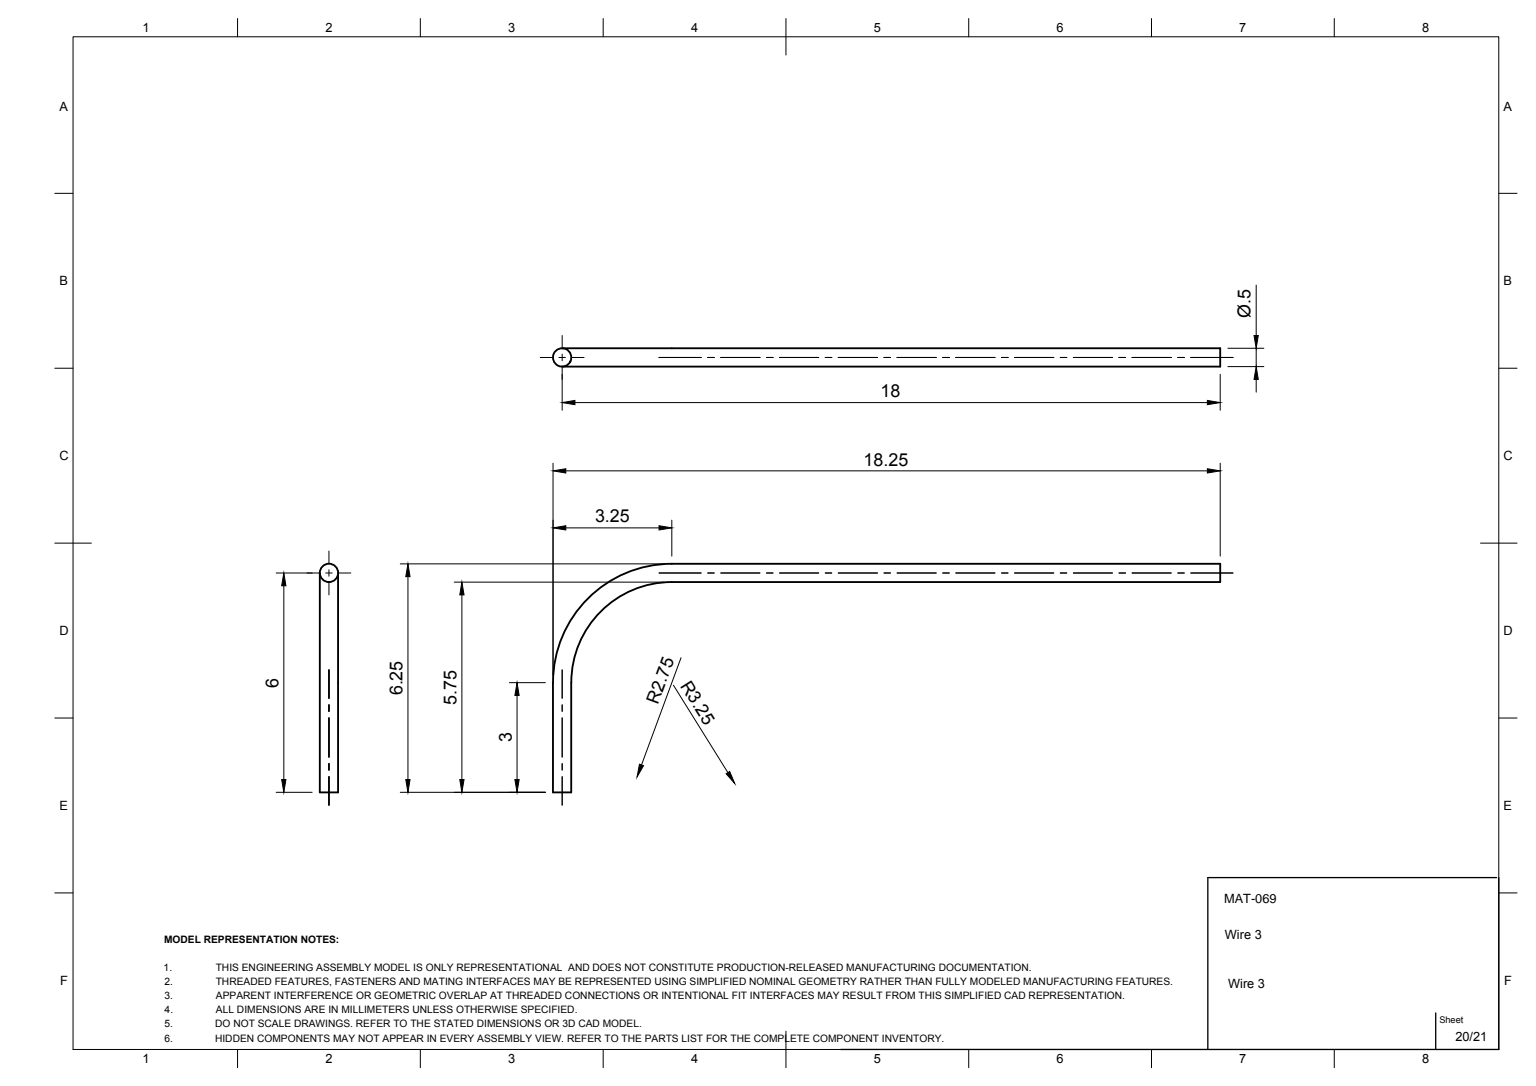
ISO-10303-21;
HEADER;
/* Generated by software containing ST-Developer
 * from STEP Tools, Inc. (www.steptools.com) 
 */

FILE_DESCRIPTION(
/* description */ ('CAx-IF Rec.Pracs.---Representation and Presentation of Product Manufa
cturing Information (PMI)---4.0---2014-10-13'),
/* implementation_level */ '2;1');

FILE_NAME(
/* name */ 'Wire 3.step',
/* time_stamp */ '2026-10-24T15:08:39-07:00',
/* author */ (''),
/* organization */ (''),
/* preprocessor_version */ 'ST-DEVELOPER v20.2',
/* originating_system */ 'Autodesk Translation Framework v15.17.0.0',
/* authorisation */ '');

FILE_SCHEMA (('AP242_MANAGED_MODEL_BASED_3D_ENGINEERING_MIM_LF { 1 0 10303 442 2 1 4 }'));
ENDSEC;

DATA;
#10=MECHANICAL_DESIGN_GEOMETRIC_PRESENTATION_REPRESENTATION('',(#838),#50081);
#779=TOROIDAL_SURFACE('',#10984,0.003,0.00025);
#798=SHAPE_REPRESENTATION_RELATIONSHIP('SRR','None',#50166,#818);
#818=ADVANCED_BREP_SHAPE_REPRESENTATION('',(#858),#50079);
#838=STYLED_ITEM('',(#50260),#858);
#858=MANIFOLD_SOLID_BREP('Body1',#9883);
#1097=PLANE('',#10990);
#1098=PLANE('',#10991);
#1625=FACE_OUTER_BOUND('',#2223,.T.);
#1626=FACE_OUTER_BOUND('',#2224,.T.);
#1627=FACE_OUTER_BOUND('',#2225,.T.);
#1628=FACE_OUTER_BOUND('',#2226,.T.);
#1629=FACE_OUTER_BOUND('',#2227,.T.);
#2223=EDGE_LOOP('',(#9060,#9061,#9062,#9063,#9064));
#2224=EDGE_LOOP('',(#9065,#9066,#9067,#9068,#9069,#9070));
#2225=EDGE_LOOP('',(#9071,#9072,#9073,#9074,#9075));
#2226=EDGE_LOOP('',(#9076));
#2227=EDGE_LOOP('',(#9077));
#2813=LINE('',#49284,#3391);
#2814=LINE('',#49296,#3392);
#3391=VECTOR('',#13357,0.00025);
#3392=VECTOR('',#13372,0.00025);
#3754=CIRCLE('',#10981,0.00025000000001);
#3755=CIRCLE('',#10982,0.00025000000001);
#3756=CIRCLE('',#10983,0.00025000000001);
#3757=CIRCLE('',#10985,0.00275);
#3758=CIRCLE('',#10986,0.00025000000001);
#3759=CIRCLE('',#10987,0.00025000000001);
#3760=CIRCLE('',#10989,0.00025000000001);
#4737=VERTEX_POINT('',#49281);
#4738=VERTEX_POINT('',#49283);
#4739=VERTEX_POINT('',#49285);
#4740=VERTEX_POINT('',#49289);
#4741=VERTEX_POINT('',#49291);
#4742=VERTEX_POINT('',#49295);
#6183=EDGE_CURVE('',#4737,#4737,#3754,.T.);
#6184=EDGE_CURVE('',#4737,#4738,#2813,.T.);
#6185=EDGE_CURVE('',#4738,#4739,#3755,.T.);
#6186=EDGE_CURVE('',#4739,#4738,#3756,.T.);
#6187=EDGE_CURVE('',#4739,#4740,#3757,.T.);
#6188=EDGE_CURVE('',#4740,#4741,#3758,.T.);
#6189=EDGE_CURVE('',#4741,#4740,#3759,.T.);
#6190=EDGE_CURVE('',#4741,#4742,#2814,.T.);
#6191=EDGE_CURVE('',#4742,#4742,#3760,.T.);
#9060=ORIENTED_EDGE('',*,*,#6183,.F.);
#9061=ORIENTED_EDGE('',*,*,#6184,.T.);
#9062=ORIENTED_EDGE('',*,*,#6185,.T.);
#9063=ORIENTED_EDGE('',*,*,#6186,.T.);
#9064=ORIENTED_EDGE('',*,*,#6184,.F.);
#9065=ORIENTED_EDGE('',*,*,#6186,.F.);
#9066=ORIENTED_EDGE('',*,*,#6187,.T.);
#9067=ORIENTED_EDGE('',*,*,#6188,.T.);
#9068=ORIENTED_EDGE('',*,*,#6189,.T.);
#9069=ORIENTED_EDGE('',*,*,#6187,.F.);
#9070=ORIENTED_EDGE('',*,*,#6185,.F.);
#9071=ORIENTED_EDGE('',*,*,#6189,.F.);
#9072=ORIENTED_EDGE('',*,*,#6190,.T.);
#9073=ORIENTED_EDGE('',*,*,#6191,.T.);
#9074=ORIENTED_EDGE('',*,*,#6190,.F.);
#9075=ORIENTED_EDGE('',*,*,#6188,.F.);
#9076=ORIENTED_EDGE('',*,*,#6183,.T.);
#9077=ORIENTED_EDGE('',*,*,#6191,.F.);
#9317=CYLINDRICAL_SURFACE('',#10980,0.00025);
#9318=CYLINDRICAL_SURFACE('',#10988,0.00025);
#9847=ADVANCED_FACE('',(#1625),#9317,.T.);
#9848=ADVANCED_FACE('',(#1626),#779,.T.);
#9849=ADVANCED_FACE('',(#1627),#9318,.T.);
#9850=ADVANCED_FACE('',(#1628),#1097,.T.);
#9851=ADVANCED_FACE('',(#1629),#1098,.F.);
#9883=CLOSED_SHELL('',(#9847,#9848,#9849,#9850,#9851));
#10979=AXIS2_PLACEMENT_3D('',#49279,#13351,#13352);
#10980=AXIS2_PLACEMENT_3D('',#49280,#13353,#13354);
#10981=AXIS2_PLACEMENT_3D('',#49282,#13355,#13356);
#10982=AXIS2_PLACEMENT_3D('',#49286,#13358,#13359);
#10983=AXIS2_PLACEMENT_3D('',#49287,#13360,#13361);
#10984=AXIS2_PLACEMENT_3D('',#49288,#13362,#13363);
#10985=AXIS2_PLACEMENT_3D('',#49290,#13364,#13365);
#10986=AXIS2_PLACEMENT_3D('',#49292,#13366,#13367);
#10987=AXIS2_PLACEMENT_3D('',#49293,#13368,#13369);
#10988=AXIS2_PLACEMENT_3D('',#49294,#13370,#13371);
#10989=AXIS2_PLACEMENT_3D('',#49297,#13373,#13374);
#10990=AXIS2_PLACEMENT_3D('',#49298,#13375,#13376);
#10991=AXIS2_PLACEMENT_3D('',#49299,#13377,#13378);
#13351=DIRECTION('axis',(0.,0.,1.));
#13352=DIRECTION('refdir',(1.,0.,0.));
#13353=DIRECTION('center_axis',(2.42833204006769E-16,2.41473507855972E-15,
-1.));
#13354=DIRECTION('ref_axis',(0.422618261740706,0.906307787036647,2.29111895189949E-15));
#13355=DIRECTION('center_axis',(3.62526098085663E-11,-1.69023416117786E-11,
-1.));
#13356=DIRECTION('ref_axis',(0.422618261740706,0.906307787036647,2.29111895186089E-15));
#13357=DIRECTION('',(-2.42833204006769E-16,-2.41473507855972E-15,1.));
#13358=DIRECTION('center_axis',(3.62526098085663E-11,-1.69023416117786E-11,
-1.));
#13359=DIRECTION('ref_axis',(0.422618261740706,0.906307787036647,2.29111895186089E-15));
#13360=DIRECTION('center_axis',(3.62526098085663E-11,-1.69023416117786E-11,
-1.));
#13361=DIRECTION('ref_axis',(0.422618261740706,0.906307787036647,2.29111895186089E-15));
#13362=DIRECTION('center_axis',(0.422618261740706,0.906307787036647,1.97116866169388E-15));
#13363=DIRECTION('ref_axis',(1.33440267382831E-16,2.1350442781253E-15,-1.));
#13364=DIRECTION('center_axis',(-0.422618261740706,-0.906307787036647,-1.97116866169388E-15));
#13365=DIRECTION('ref_axis',(3.8032634610719E-16,1.99759488807599E-15,-1.));
#13366=DIRECTION('center_axis',(0.906307787036647,-0.422618261740706,-8.00429517722823E-16));
#13367=DIRECTION('ref_axis',(0.422618261740706,0.906307787036647,1.97116866169388E-15));
#13368=DIRECTION('center_axis',(0.906307787036647,-0.422618261740706,-8.00429517722823E-16));
#13369=DIRECTION('ref_axis',(0.422618261740706,0.906307787036647,1.97116866169388E-15));
#13370=DIRECTION('center_axis',(0.906307787036647,-0.422618261740706,-8.00429517722823E-16));
#13371=DIRECTION('ref_axis',(0.422618261740706,0.906307787036647,1.97116866169388E-15));
#13372=DIRECTION('',(-0.906307787036647,0.422618261740706,8.00429517722823E-16));
#13373=DIRECTION('center_axis',(0.906307787036647,-0.422618261740706,-8.00429517722823E-16));
#13374=DIRECTION('ref_axis',(0.422618261740706,0.906307787036647,1.97116866169388E-15));
#13375=DIRECTION('center_axis',(2.98328550528607E-16,2.38885717348462E-15,
-1.));
#13376=DIRECTION('ref_axis',(0.906307787036647,-0.422618261740706,-7.39197177765454E-16));
#13377=DIRECTION('center_axis',(0.906307787036647,-0.422618261740706,-8.00429517722823E-16));
#13378=DIRECTION('ref_axis',(2.42833204006769E-16,2.41473507855972E-15,
-1.));
#49279=CARTESIAN_POINT('',(0.,0.,0.));
#49280=CARTESIAN_POINT('Origin',(0.00621130913087035,-0.035075620496354,
-0.0013758532865581));
#49281=CARTESIAN_POINT('',(0.00610565456543517,-0.0353021974431132,-0.0043758532865581));
#49282=CARTESIAN_POINT('Origin',(0.00621130913087458,-0.035075620496345,
-0.0043758532865481));
#49283=CARTESIAN_POINT('',(0.00610565456543517,-0.0353021974431132,-0.0013758532865381));
#49284=CARTESIAN_POINT('',(0.00610565456543517,-0.0353021974431132,-0.0013758532865581));
#49285=CARTESIAN_POINT('',(0.00598473218410215,-0.0349699659309146,-0.0013758532865581));
#49286=CARTESIAN_POINT('Origin',(0.00621130913087458,-0.035075620496345,
-0.0013758532865481));
#49287=CARTESIAN_POINT('Origin',(0.00621130913087458,-0.035075620496345,
-0.0013758532865481));
#49288=CARTESIAN_POINT('Origin',(0.00349238576976041,-0.0338077657111319,
-0.0013758532865581));
#49289=CARTESIAN_POINT('',(0.00349238576975134,-0.0338077657111277,0.0013741467134419));
#49290=CARTESIAN_POINT('Origin',(0.00349238576976041,-0.0338077657111319,
-0.0013758532865581));
#49291=CARTESIAN_POINT('',(0.00338673120431614,-0.0340343426578869,0.0016241467134419));
#49292=CARTESIAN_POINT('Origin',(0.00349238576975557,-0.0338077657111186,
0.0016241467134519));
#49293=CARTESIAN_POINT('Origin',(0.00349238576975557,-0.0338077657111186,
0.0016241467134519));
#49294=CARTESIAN_POINT('Origin',(-0.0101022310357893,-0.0274684917850214,
0.00162414671344191));
#49295=CARTESIAN_POINT('',(-0.0102078856012336,-0.0276950687317763,0.00162414671344191));
#49296=CARTESIAN_POINT('',(-0.0102078856012245,-0.0276950687317806,0.00162414671344191));
#49297=CARTESIAN_POINT('Origin',(-0.0101022310357941,-0.027468491785008,
0.00162414671345191));
#49298=CARTESIAN_POINT('Origin',(0.00621130913087035,-0.035075620496354,
-0.0043758532865581));
#49299=CARTESIAN_POINT('Origin',(-0.0101022310357893,-0.0274684917850214,
0.00162414671344191));
#50057=UNCERTAINTY_MEASURE_WITH_UNIT(LENGTH_MEASURE(1.E-5),#50082,
'DISTANCE_ACCURACY_VALUE',
'Maximum model space distance between geometric entities at asserted c
onnectivities');
#50059=UNCERTAINTY_MEASURE_WITH_UNIT(LENGTH_MEASURE(1.E-5),#50082,
'DISTANCE_ACCURACY_VALUE',
'Maximum model space distance between geometric entities at asserted c
onnectivities');
#50079=(
GEOMETRIC_REPRESENTATION_CONTEXT(3)
GLOBAL_UNCERTAINTY_ASSIGNED_CONTEXT((#50057))
GLOBAL_UNIT_ASSIGNED_CONTEXT((#50082,#50083,#50084))
REPRESENTATION_CONTEXT('','3D')
);
#50081=(
GEOMETRIC_REPRESENTATION_CONTEXT(3)
GLOBAL_UNCERTAINTY_ASSIGNED_CONTEXT((#50059))
GLOBAL_UNIT_ASSIGNED_CONTEXT((#50082,#50083,#50084))
REPRESENTATION_CONTEXT('','3D')
);
#50082=(
LENGTH_UNIT()
NAMED_UNIT(*)
SI_UNIT($,.METRE.)
);
#50083=(
NAMED_UNIT(*)
PLANE_ANGLE_UNIT()
SI_UNIT($,.RADIAN.)
);
#50084=(
NAMED_UNIT(*)
SI_UNIT($,.STERADIAN.)
SOLID_ANGLE_UNIT()
);
#50104=SHAPE_DEFINITION_REPRESENTATION(#50125,#50166);
#50125=PRODUCT_DEFINITION_SHAPE('',$,#50188);
#50166=SHAPE_REPRESENTATION('',(#10979),#50079);
#50168=PRODUCT_DEFINITION_CONTEXT('part definition',#50233,'design');
#50188=PRODUCT_DEFINITION('Wire 3','Wire 3',#50209,#50168);
#50209=PRODUCT_DEFINITION_FORMATION('',$,#50254);
#50233=APPLICATION_CONTEXT('Managed model based 3d engineering');
#50234=PRODUCT_CONTEXT('part definition',#50233,'mechanical');
#50254=PRODUCT('Wire 3','Wire 3','Sensor Cartridge v1',(#50234));
#50260=PRESENTATION_STYLE_ASSIGNMENT((#50267));
#50267=SURFACE_STYLE_USAGE(.BOTH.,#50274);
#50274=SURFACE_SIDE_STYLE('',(#50281));
#50281=SURFACE_STYLE_FILL_AREA(#50288);
#50288=FILL_AREA_STYLE('Opaque(25,25,25)',(#50295));
#50295=FILL_AREA_STYLE_COLOUR('Opaque(25,25,25)',#50302);
#50302=COLOUR_RGB('Opaque(25,25,25)',0.0980392156862745,0.0980392156862745,
0.0980392156862745);
ENDSEC;
END-ISO-10303-21;
